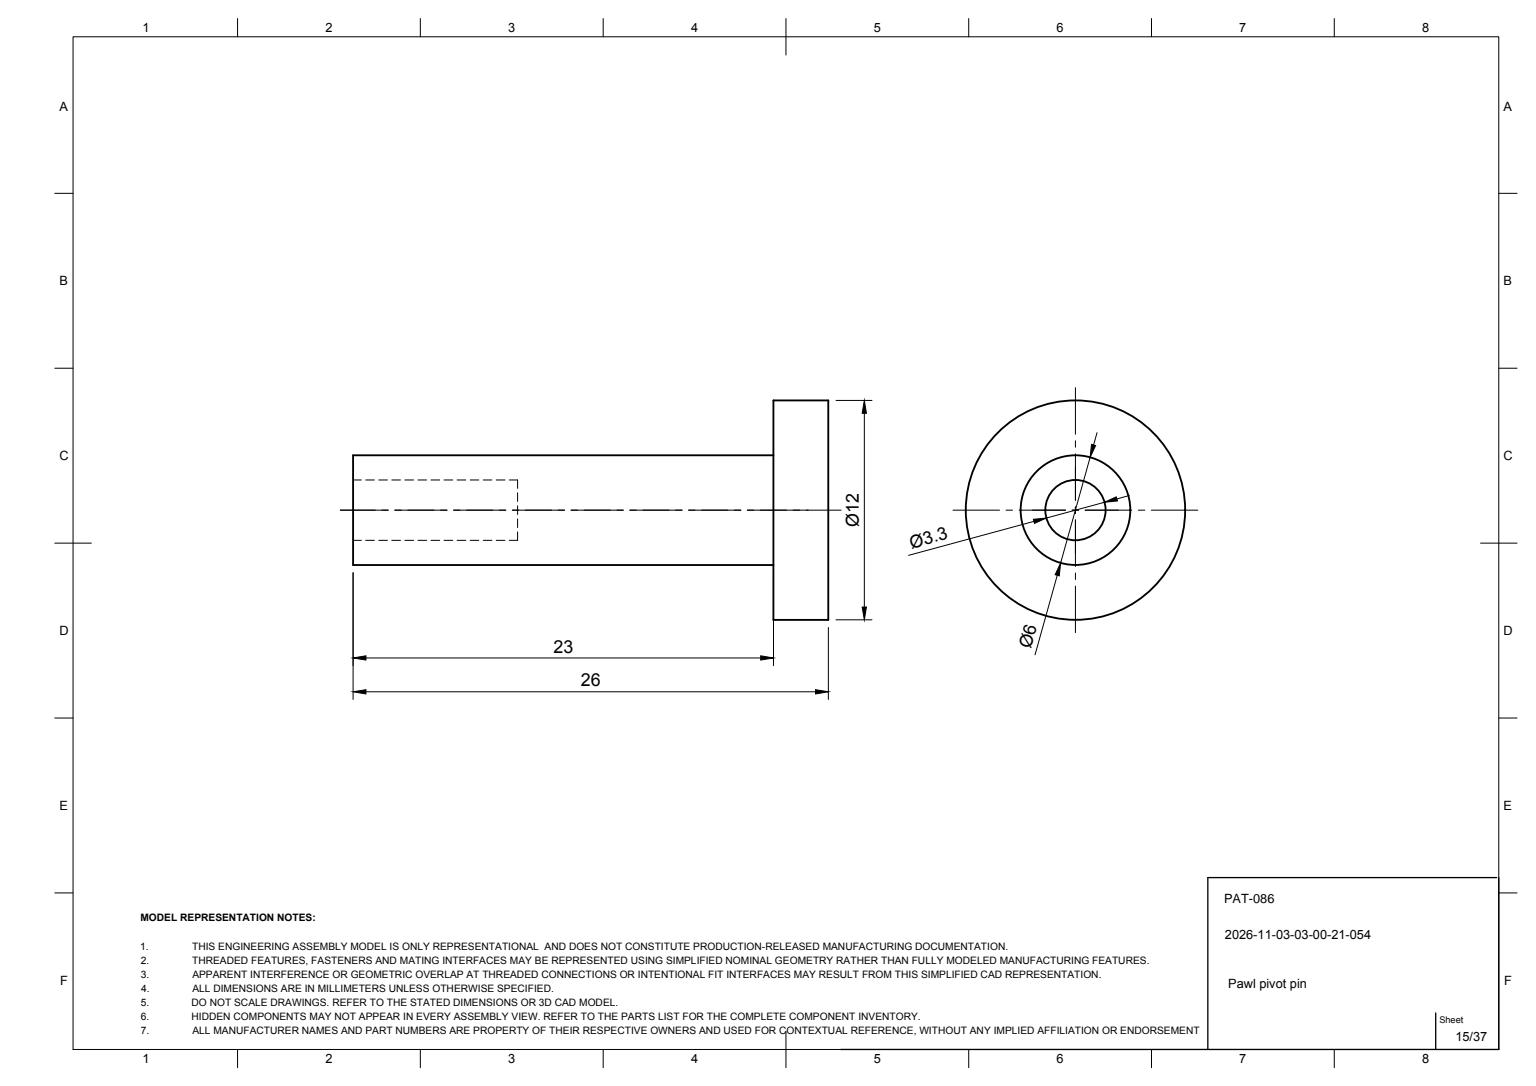
ISO-10303-21;
HEADER;
/* Generated by software containing ST-Developer
 * from STEP Tools, Inc. (www.steptools.com) 
 */

FILE_DESCRIPTION(
/* description */ ('Ratchet and pawl hand winch drum'),
/* implementation_level */ '2;1');

FILE_NAME(
/* name */ 'Pawl pivot pin.step',
/* time_stamp */ '2026-10-27T12:42:58-07:00',
/* author */ (''),
/* organization */ (''),
/* preprocessor_version */ 'ST-DEVELOPER v20.2',
/* originating_system */ 'Autodesk Translation Framework v15.17.0.0',
/* authorisation */ '');

FILE_SCHEMA (('AUTOMOTIVE_DESIGN { 1 0 10303 214 3 1 1 }'));
ENDSEC;

DATA;
#10=MECHANICAL_DESIGN_GEOMETRIC_PRESENTATION_REPRESENTATION('',(#399),#11801);
#331=SHAPE_REPRESENTATION_RELATIONSHIP('SRR','None',#11957,#365);
#365=ADVANCED_BREP_SHAPE_REPRESENTATION('',(#434),#11774);
#399=STYLED_ITEM('',(#12213),#434);
#434=MANIFOLD_SOLID_BREP('Body1',#6276);
#523=FACE_BOUND('',#1364,.T.);
#524=FACE_BOUND('',#1369,.T.);
#658=PLANE('',#6875);
#659=PLANE('',#6876);
#660=PLANE('',#6881);
#661=PLANE('',#6884);
#938=FACE_OUTER_BOUND('',#1361,.T.);
#939=FACE_OUTER_BOUND('',#1362,.T.);
#940=FACE_OUTER_BOUND('',#1363,.T.);
#941=FACE_OUTER_BOUND('',#1365,.T.);
#942=FACE_OUTER_BOUND('',#1366,.T.);
#943=FACE_OUTER_BOUND('',#1367,.T.);
#944=FACE_OUTER_BOUND('',#1368,.T.);
#1361=EDGE_LOOP('',(#4661,#4662,#4663,#4664));
#1362=EDGE_LOOP('',(#4665));
#1363=EDGE_LOOP('',(#4666));
#1364=EDGE_LOOP('',(#4667));
#1365=EDGE_LOOP('',(#4668,#4669,#4670,#4671));
#1366=EDGE_LOOP('',(#4672));
#1367=EDGE_LOOP('',(#4673,#4674,#4675,#4676));
#1368=EDGE_LOOP('',(#4677));
#1369=EDGE_LOOP('',(#4678));
#1822=LINE('',#9687,#2333);
#1823=LINE('',#9697,#2334);
#1824=LINE('',#9703,#2335);
#2333=VECTOR('',#7873,0.165);
#2334=VECTOR('',#7886,0.6);
#2335=VECTOR('',#7895,0.3);
#2801=CIRCLE('',#6873,0.165);
#2802=CIRCLE('',#6874,0.165);
#2803=CIRCLE('',#6877,0.6);
#2804=CIRCLE('',#6878,0.3);
#2805=CIRCLE('',#6880,0.6);
#2806=CIRCLE('',#6883,0.3);
#3080=VERTEX_POINT('',#9684);
#3081=VERTEX_POINT('',#9686);
#3082=VERTEX_POINT('',#9691);
#3083=VERTEX_POINT('',#9693);
#3084=VERTEX_POINT('',#9696);
#3085=VERTEX_POINT('',#9701);
#3674=EDGE_CURVE('',#3080,#3080,#2801,.T.);
#3675=EDGE_CURVE('',#3080,#3081,#1822,.T.);
#3676=EDGE_CURVE('',#3081,#3081,#2802,.T.);
#3677=EDGE_CURVE('',#3082,#3082,#2803,.T.);
#3678=EDGE_CURVE('',#3083,#3083,#2804,.T.);
#3679=EDGE_CURVE('',#3082,#3084,#1823,.T.);
#3680=EDGE_CURVE('',#3084,#3084,#2805,.T.);
#3681=EDGE_CURVE('',#3085,#3085,#2806,.T.);
#3682=EDGE_CURVE('',#3085,#3083,#1824,.T.);
#4661=ORIENTED_EDGE('',*,*,#3674,.F.);
#4662=ORIENTED_EDGE('',*,*,#3675,.T.);
#4663=ORIENTED_EDGE('',*,*,#3676,.F.);
#4664=ORIENTED_EDGE('',*,*,#3675,.F.);
#4665=ORIENTED_EDGE('',*,*,#3674,.T.);
#4666=ORIENTED_EDGE('',*,*,#3677,.T.);
#4667=ORIENTED_EDGE('',*,*,#3678,.F.);
#4668=ORIENTED_EDGE('',*,*,#3677,.F.);
#4669=ORIENTED_EDGE('',*,*,#3679,.T.);
#4670=ORIENTED_EDGE('',*,*,#3680,.T.);
#4671=ORIENTED_EDGE('',*,*,#3679,.F.);
#4672=ORIENTED_EDGE('',*,*,#3680,.F.);
#4673=ORIENTED_EDGE('',*,*,#3681,.F.);
#4674=ORIENTED_EDGE('',*,*,#3682,.T.);
#4675=ORIENTED_EDGE('',*,*,#3678,.T.);
#4676=ORIENTED_EDGE('',*,*,#3682,.F.);
#4677=ORIENTED_EDGE('',*,*,#3681,.T.);
#4678=ORIENTED_EDGE('',*,*,#3676,.T.);
#5848=CYLINDRICAL_SURFACE('',#6872,0.165);
#5849=CYLINDRICAL_SURFACE('',#6879,0.6);
#5850=CYLINDRICAL_SURFACE('',#6882,0.3);
#6008=ADVANCED_FACE('',(#938),#5848,.F.);
#6009=ADVANCED_FACE('',(#939),#658,.T.);
#6010=ADVANCED_FACE('',(#940,#523),#659,.T.);
#6011=ADVANCED_FACE('',(#941),#5849,.T.);
#6012=ADVANCED_FACE('',(#942),#660,.F.);
#6013=ADVANCED_FACE('',(#943),#5850,.T.);
#6014=ADVANCED_FACE('',(#944,#524),#661,.T.);
#6276=CLOSED_SHELL('',(#6008,#6009,#6010,#6011,#6012,#6013,#6014));
#6871=AXIS2_PLACEMENT_3D('',#9682,#7867,#7868);
#6872=AXIS2_PLACEMENT_3D('',#9683,#7869,#7870);
#6873=AXIS2_PLACEMENT_3D('',#9685,#7871,#7872);
#6874=AXIS2_PLACEMENT_3D('',#9688,#7874,#7875);
#6875=AXIS2_PLACEMENT_3D('',#9689,#7876,#7877);
#6876=AXIS2_PLACEMENT_3D('',#9690,#7878,#7879);
#6877=AXIS2_PLACEMENT_3D('',#9692,#7880,#7881);
#6878=AXIS2_PLACEMENT_3D('',#9694,#7882,#7883);
#6879=AXIS2_PLACEMENT_3D('',#9695,#7884,#7885);
#6880=AXIS2_PLACEMENT_3D('',#9698,#7887,#7888);
#6881=AXIS2_PLACEMENT_3D('',#9699,#7889,#7890);
#6882=AXIS2_PLACEMENT_3D('',#9700,#7891,#7892);
#6883=AXIS2_PLACEMENT_3D('',#9702,#7893,#7894);
#6884=AXIS2_PLACEMENT_3D('',#9704,#7896,#7897);
#7867=DIRECTION('axis',(0.,0.,1.));
#7868=DIRECTION('refdir',(1.,0.,0.));
#7869=DIRECTION('center_axis',(0.,1.,0.));
#7870=DIRECTION('ref_axis',(1.,0.,0.));
#7871=DIRECTION('center_axis',(0.,1.,0.));
#7872=DIRECTION('ref_axis',(1.,0.,0.));
#7873=DIRECTION('',(0.,1.,0.));
#7874=DIRECTION('center_axis',(0.,-1.,0.));
#7875=DIRECTION('ref_axis',(1.,0.,0.));
#7876=DIRECTION('center_axis',(0.,1.,0.));
#7877=DIRECTION('ref_axis',(1.,0.,0.));
#7878=DIRECTION('center_axis',(0.,1.,0.));
#7879=DIRECTION('ref_axis',(1.,0.,0.));
#7880=DIRECTION('center_axis',(0.,1.,0.));
#7881=DIRECTION('ref_axis',(1.,0.,0.));
#7882=DIRECTION('center_axis',(0.,1.,0.));
#7883=DIRECTION('ref_axis',(1.,0.,0.));
#7884=DIRECTION('center_axis',(0.,1.,0.));
#7885=DIRECTION('ref_axis',(1.,0.,0.));
#7886=DIRECTION('',(0.,-1.,0.));
#7887=DIRECTION('center_axis',(0.,1.,0.));
#7888=DIRECTION('ref_axis',(1.,0.,0.));
#7889=DIRECTION('center_axis',(0.,1.,0.));
#7890=DIRECTION('ref_axis',(1.,0.,0.));
#7891=DIRECTION('center_axis',(0.,1.,0.));
#7892=DIRECTION('ref_axis',(1.,0.,0.));
#7893=DIRECTION('center_axis',(0.,1.,0.));
#7894=DIRECTION('ref_axis',(1.,0.,0.));
#7895=DIRECTION('',(0.,-1.,0.));
#7896=DIRECTION('center_axis',(0.,1.,0.));
#7897=DIRECTION('ref_axis',(1.,0.,0.));
#9682=CARTESIAN_POINT('',(0.,0.,0.));
#9683=CARTESIAN_POINT('Origin',(6.5,-3.8,10.));
#9684=CARTESIAN_POINT('',(6.335,-3.8,10.));
#9685=CARTESIAN_POINT('Origin',(6.5,-3.8,10.));
#9686=CARTESIAN_POINT('',(6.335,-2.9,10.));
#9687=CARTESIAN_POINT('',(6.335,-3.8,10.));
#9688=CARTESIAN_POINT('Origin',(6.5,-2.9,10.));
#9689=CARTESIAN_POINT('Origin',(6.5,-3.8,10.));
#9690=CARTESIAN_POINT('Origin',(6.5,-5.2,10.));
#9691=CARTESIAN_POINT('',(5.9,-5.2,10.));
#9692=CARTESIAN_POINT('Origin',(6.5,-5.2,10.));
#9693=CARTESIAN_POINT('',(6.2,-5.2,10.));
#9694=CARTESIAN_POINT('Origin',(6.5,-5.2,10.));
#9695=CARTESIAN_POINT('Origin',(6.5,-5.5,10.));
#9696=CARTESIAN_POINT('',(5.9,-5.5,10.));
#9697=CARTESIAN_POINT('',(5.9,-5.5,10.));
#9698=CARTESIAN_POINT('Origin',(6.5,-5.5,10.));
#9699=CARTESIAN_POINT('Origin',(6.5,-5.5,10.));
#9700=CARTESIAN_POINT('Origin',(6.5,-5.2,10.));
#9701=CARTESIAN_POINT('',(6.2,-2.9,10.));
#9702=CARTESIAN_POINT('Origin',(6.5,-2.9,10.));
#9703=CARTESIAN_POINT('',(6.2,-5.2,10.));
#9704=CARTESIAN_POINT('Origin',(6.5,-2.9,10.));
#11734=UNCERTAINTY_MEASURE_WITH_UNIT(LENGTH_MEASURE(0.001),#11802,
'DISTANCE_ACCURACY_VALUE',
'Maximum model space distance between geometric entities at asserted c
onnectivities');
#11761=UNCERTAINTY_MEASURE_WITH_UNIT(LENGTH_MEASURE(0.001),#11802,
'DISTANCE_ACCURACY_VALUE',
'Maximum model space distance between geometric entities at asserted c
onnectivities');
#11774=(
GEOMETRIC_REPRESENTATION_CONTEXT(3)
GLOBAL_UNCERTAINTY_ASSIGNED_CONTEXT((#11734))
GLOBAL_UNIT_ASSIGNED_CONTEXT((#11802,#11804,#11805))
REPRESENTATION_CONTEXT('','3D')
);
#11801=(
GEOMETRIC_REPRESENTATION_CONTEXT(3)
GLOBAL_UNCERTAINTY_ASSIGNED_CONTEXT((#11761))
GLOBAL_UNIT_ASSIGNED_CONTEXT((#11802,#11804,#11805))
REPRESENTATION_CONTEXT('','3D')
);
#11802=(
LENGTH_UNIT()
NAMED_UNIT(*)
SI_UNIT(.CENTI.,.METRE.)
);
#11804=(
NAMED_UNIT(*)
PLANE_ANGLE_UNIT()
SI_UNIT($,.RADIAN.)
);
#11805=(
NAMED_UNIT(*)
SI_UNIT($,.STERADIAN.)
SOLID_ANGLE_UNIT()
);
#11818=SHAPE_DEFINITION_REPRESENTATION(#11857,#11957);
#11857=PRODUCT_DEFINITION_SHAPE('',$,#11997);
#11957=SHAPE_REPRESENTATION('',(#6871),#11774);
#11984=PRODUCT_DEFINITION_CONTEXT('part definition',#12103,'design');
#11997=PRODUCT_DEFINITION('Pawl pivot pin','Pawl pivot pin',#12036,#11984);
#12036=PRODUCT_DEFINITION_FORMATION('',$,#12117);
#12103=APPLICATION_CONTEXT(
'Core Data for Automotive Mechanical Design Process');
#12104=PRODUCT_CONTEXT('part definition',#12103,'mechanical');
#12117=PRODUCT('Pawl pivot pin','Pawl pivot pin','Pawl pivot pin',(#12104));
#12207=COLOUR_RGB('Grey',0.48,0.52,0.57);
#12208=FILL_AREA_STYLE_COLOUR('',#12207);
#12209=FILL_AREA_STYLE('',(#12208));
#12210=SURFACE_STYLE_FILL_AREA(#12209);
#12211=SURFACE_SIDE_STYLE('',(#12210));
#12212=SURFACE_STYLE_USAGE(.BOTH.,#12211);
#12213=PRESENTATION_STYLE_ASSIGNMENT((#12212));
ENDSEC;
END-ISO-10303-21;
